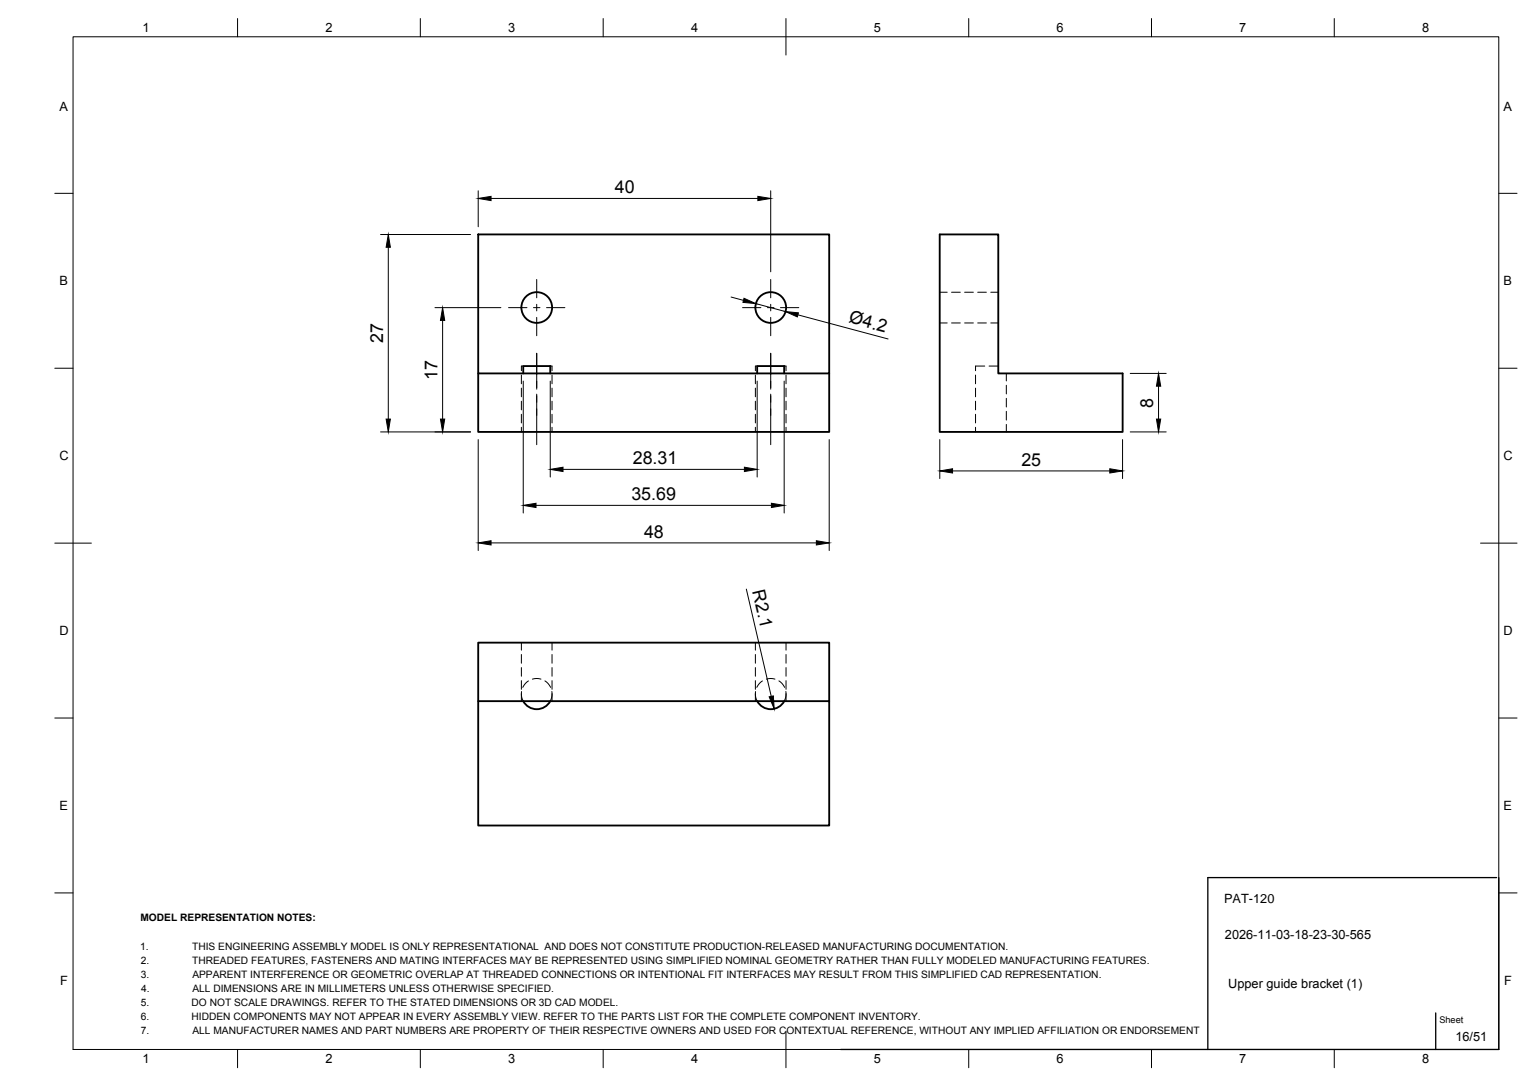
ISO-10303-21;
HEADER;
/* Generated by software containing ST-Developer
 * from STEP Tools, Inc. (www.steptools.com) 
 */

FILE_DESCRIPTION(
/* description */ ('Vibration shaker table dummy'),
/* implementation_level */ '2;1');

FILE_NAME(
/* name */ 'Upper guide bracket (1).step',
/* time_stamp */ '2026-10-27T10:55:14-07:00',
/* author */ (''),
/* organization */ (''),
/* preprocessor_version */ 'ST-DEVELOPER v20.2',
/* originating_system */ 'Autodesk Translation Framework v15.17.0.0',
/* authorisation */ '');

FILE_SCHEMA (('AUTOMOTIVE_DESIGN { 1 0 10303 214 3 1 1 }'));
ENDSEC;

DATA;
#10=MECHANICAL_DESIGN_GEOMETRIC_PRESENTATION_REPRESENTATION('',(#697),#22394);
#605=SHAPE_REPRESENTATION_RELATIONSHIP('SRR','None',#22651,#651);
#651=ADVANCED_BREP_SHAPE_REPRESENTATION('',(#743),#22357);
#697=STYLED_ITEM('',(#22940),#743);
#743=MANIFOLD_SOLID_BREP('Body1',#9215);
#883=FACE_BOUND('',#2092,.T.);
#884=FACE_BOUND('',#2093,.T.);
#885=FACE_BOUND('',#2097,.T.);
#886=FACE_BOUND('',#2098,.T.);
#887=FACE_BOUND('',#2101,.T.);
#888=FACE_BOUND('',#2102,.T.);
#1134=PLANE('',#10051);
#1135=PLANE('',#10057);
#1136=PLANE('',#10058);
#1137=PLANE('',#10059);
#1138=PLANE('',#10060);
#1139=PLANE('',#10061);
#1140=PLANE('',#10062);
#1141=PLANE('',#10063);
#1142=PLANE('',#10064);
#1143=PLANE('',#10065);
#1478=FACE_OUTER_BOUND('',#2084,.T.);
#1479=FACE_OUTER_BOUND('',#2085,.T.);
#1480=FACE_OUTER_BOUND('',#2086,.T.);
#1481=FACE_OUTER_BOUND('',#2087,.T.);
#1482=FACE_OUTER_BOUND('',#2088,.T.);
#1483=FACE_OUTER_BOUND('',#2089,.T.);
#1484=FACE_OUTER_BOUND('',#2090,.T.);
#1485=FACE_OUTER_BOUND('',#2091,.T.);
#1486=FACE_OUTER_BOUND('',#2094,.T.);
#1487=FACE_OUTER_BOUND('',#2095,.T.);
#1488=FACE_OUTER_BOUND('',#2096,.T.);
#1489=FACE_OUTER_BOUND('',#2099,.T.);
#1490=FACE_OUTER_BOUND('',#2100,.T.);
#1491=FACE_OUTER_BOUND('',#2103,.T.);
#2084=EDGE_LOOP('',(#6876,#6877,#6878,#6879));
#2085=EDGE_LOOP('',(#6880,#6881,#6882,#6883));
#2086=EDGE_LOOP('',(#6884,#6885,#6886,#6887,#6888,#6889,#6890,#6891));
#2087=EDGE_LOOP('',(#6892,#6893,#6894));
#2088=EDGE_LOOP('',(#6895,#6896,#6897,#6898,#6899,#6900,#6901,#6902));
#2089=EDGE_LOOP('',(#6903,#6904,#6905));
#2090=EDGE_LOOP('',(#6906,#6907,#6908,#6909,#6910,#6911,#6912,#6913));
#2091=EDGE_LOOP('',(#6914,#6915,#6916,#6917,#6918,#6919,#6920,#6921,#6922,
#6923,#6924,#6925));
#2092=EDGE_LOOP('',(#6926));
#2093=EDGE_LOOP('',(#6927));
#2094=EDGE_LOOP('',(#6928,#6929,#6930,#6931));
#2095=EDGE_LOOP('',(#6932,#6933,#6934,#6935,#6936,#6937));
#2096=EDGE_LOOP('',(#6938,#6939,#6940,#6941));
#2097=EDGE_LOOP('',(#6942));
#2098=EDGE_LOOP('',(#6943));
#2099=EDGE_LOOP('',(#6944,#6945,#6946,#6947,#6948,#6949));
#2100=EDGE_LOOP('',(#6950,#6951,#6952,#6953));
#2101=EDGE_LOOP('',(#6954));
#2102=EDGE_LOOP('',(#6955));
#2103=EDGE_LOOP('',(#6956,#6957,#6958,#6959));
#2806=LINE('',#16101,#3425);
#2807=LINE('',#16107,#3426);
#2808=LINE('',#16113,#3427);
#2809=LINE('',#16117,#3428);
#2810=LINE('',#16121,#3429);
#2811=LINE('',#16124,#3430);
#2812=LINE('',#16129,#3431);
#2813=LINE('',#16133,#3432);
#2814=LINE('',#16137,#3433);
#2815=LINE('',#16140,#3434);
#2816=LINE('',#16142,#3435);
#2817=LINE('',#16144,#3436);
#2818=LINE('',#16146,#3437);
#2819=LINE('',#16148,#3438);
#2820=LINE('',#16150,#3439);
#2821=LINE('',#16151,#3440);
#2822=LINE('',#16154,#3441);
#2823=LINE('',#16156,#3442);
#2824=LINE('',#16157,#3443);
#2825=LINE('',#16161,#3444);
#2826=LINE('',#16162,#3445);
#2827=LINE('',#16163,#3446);
#2828=LINE('',#16167,#3447);
#2829=LINE('',#16168,#3448);
#2830=LINE('',#16169,#3449);
#2831=LINE('',#16173,#3450);
#2832=LINE('',#16174,#3451);
#2833=LINE('',#16175,#3452);
#2834=LINE('',#16177,#3453);
#2835=LINE('',#16178,#3454);
#3425=VECTOR('',#11698,0.21);
#3426=VECTOR('',#11705,0.21);
#3427=VECTOR('',#11712,0.21);
#3428=VECTOR('',#11715,1.);
#3429=VECTOR('',#11718,1.);
#3430=VECTOR('',#11723,1.);
#3431=VECTOR('',#11728,0.21);
#3432=VECTOR('',#11731,1.);
#3433=VECTOR('',#11734,1.);
#3434=VECTOR('',#11739,1.);
#3435=VECTOR('',#11742,1.);
#3436=VECTOR('',#11743,1.);
#3437=VECTOR('',#11744,1.);
#3438=VECTOR('',#11745,1.);
#3439=VECTOR('',#11746,1.);
#3440=VECTOR('',#11747,1.);
#3441=VECTOR('',#11750,1.);
#3442=VECTOR('',#11751,1.);
#3443=VECTOR('',#11752,1.);
#3444=VECTOR('',#11755,1.);
#3445=VECTOR('',#11756,1.);
#3446=VECTOR('',#11757,1.);
#3447=VECTOR('',#11760,1.);
#3448=VECTOR('',#11761,1.);
#3449=VECTOR('',#11762,1.);
#3450=VECTOR('',#11765,1.);
#3451=VECTOR('',#11766,1.);
#3452=VECTOR('',#11767,1.);
#3453=VECTOR('',#11770,1.);
#3454=VECTOR('',#11771,1.);
#3990=CIRCLE('',#10041,0.21);
#3991=CIRCLE('',#10042,0.21);
#3992=CIRCLE('',#10044,0.21);
#3993=CIRCLE('',#10045,0.21);
#3994=CIRCLE('',#10047,0.21);
#3995=CIRCLE('',#10048,0.21);
#3996=CIRCLE('',#10049,0.21);
#3997=CIRCLE('',#10050,0.21);
#3998=CIRCLE('',#10053,0.21);
#3999=CIRCLE('',#10054,0.21);
#4000=CIRCLE('',#10055,0.21);
#4001=CIRCLE('',#10056,0.21);
#4577=VERTEX_POINT('',#16098);
#4578=VERTEX_POINT('',#16100);
#4579=VERTEX_POINT('',#16104);
#4580=VERTEX_POINT('',#16106);
#4581=VERTEX_POINT('',#16110);
#4582=VERTEX_POINT('',#16112);
#4583=VERTEX_POINT('',#16114);
#4584=VERTEX_POINT('',#16116);
#4585=VERTEX_POINT('',#16118);
#4586=VERTEX_POINT('',#16120);
#4587=VERTEX_POINT('',#16126);
#4588=VERTEX_POINT('',#16128);
#4589=VERTEX_POINT('',#16130);
#4590=VERTEX_POINT('',#16132);
#4591=VERTEX_POINT('',#16134);
#4592=VERTEX_POINT('',#16136);
#4593=VERTEX_POINT('',#16143);
#4594=VERTEX_POINT('',#16145);
#4595=VERTEX_POINT('',#16147);
#4596=VERTEX_POINT('',#16149);
#4597=VERTEX_POINT('',#16153);
#4598=VERTEX_POINT('',#16155);
#4599=VERTEX_POINT('',#16159);
#4600=VERTEX_POINT('',#16160);
#4601=VERTEX_POINT('',#16165);
#4602=VERTEX_POINT('',#16166);
#4603=VERTEX_POINT('',#16171);
#4604=VERTEX_POINT('',#16172);
#5431=EDGE_CURVE('',#4577,#4577,#3990,.T.);
#5432=EDGE_CURVE('',#4577,#4578,#2806,.T.);
#5433=EDGE_CURVE('',#4578,#4578,#3991,.T.);
#5434=EDGE_CURVE('',#4579,#4579,#3992,.T.);
#5435=EDGE_CURVE('',#4579,#4580,#2807,.T.);
#5436=EDGE_CURVE('',#4580,#4580,#3993,.T.);
#5437=EDGE_CURVE('',#4581,#4581,#3994,.T.);
#5438=EDGE_CURVE('',#4581,#4582,#2808,.T.);
#5439=EDGE_CURVE('',#4582,#4583,#3995,.T.);
#5440=EDGE_CURVE('',#4584,#4583,#2809,.T.);
#5441=EDGE_CURVE('',#4585,#4584,#3996,.T.);
#5442=EDGE_CURVE('',#4586,#4585,#2810,.T.);
#5443=EDGE_CURVE('',#4586,#4582,#3997,.T.);
#5444=EDGE_CURVE('',#4583,#4586,#2811,.T.);
#5445=EDGE_CURVE('',#4587,#4587,#3998,.T.);
#5446=EDGE_CURVE('',#4587,#4588,#2812,.T.);
#5447=EDGE_CURVE('',#4588,#4589,#3999,.T.);
#5448=EDGE_CURVE('',#4590,#4589,#2813,.T.);
#5449=EDGE_CURVE('',#4591,#4590,#4000,.T.);
#5450=EDGE_CURVE('',#4592,#4591,#2814,.T.);
#5451=EDGE_CURVE('',#4592,#4588,#4001,.T.);
#5452=EDGE_CURVE('',#4589,#4592,#2815,.T.);
#5453=EDGE_CURVE('',#4584,#4591,#2816,.T.);
#5454=EDGE_CURVE('',#4590,#4593,#2817,.T.);
#5455=EDGE_CURVE('',#4594,#4593,#2818,.T.);
#5456=EDGE_CURVE('',#4594,#4595,#2819,.T.);
#5457=EDGE_CURVE('',#4595,#4596,#2820,.T.);
#5458=EDGE_CURVE('',#4596,#4585,#2821,.T.);
#5459=EDGE_CURVE('',#4596,#4597,#2822,.T.);
#5460=EDGE_CURVE('',#4598,#4597,#2823,.T.);
#5461=EDGE_CURVE('',#4593,#4598,#2824,.T.);
#5462=EDGE_CURVE('',#4599,#4600,#2825,.T.);
#5463=EDGE_CURVE('',#4600,#4598,#2826,.T.);
#5464=EDGE_CURVE('',#4597,#4599,#2827,.T.);
#5465=EDGE_CURVE('',#4601,#4602,#2828,.T.);
#5466=EDGE_CURVE('',#4601,#4594,#2829,.T.);
#5467=EDGE_CURVE('',#4602,#4600,#2830,.T.);
#5468=EDGE_CURVE('',#4603,#4604,#2831,.T.);
#5469=EDGE_CURVE('',#4603,#4601,#2832,.T.);
#5470=EDGE_CURVE('',#4604,#4602,#2833,.T.);
#5471=EDGE_CURVE('',#4595,#4603,#2834,.T.);
#5472=EDGE_CURVE('',#4604,#4599,#2835,.T.);
#6876=ORIENTED_EDGE('',*,*,#5431,.F.);
#6877=ORIENTED_EDGE('',*,*,#5432,.T.);
#6878=ORIENTED_EDGE('',*,*,#5433,.F.);
#6879=ORIENTED_EDGE('',*,*,#5432,.F.);
#6880=ORIENTED_EDGE('',*,*,#5434,.F.);
#6881=ORIENTED_EDGE('',*,*,#5435,.T.);
#6882=ORIENTED_EDGE('',*,*,#5436,.F.);
#6883=ORIENTED_EDGE('',*,*,#5435,.F.);
#6884=ORIENTED_EDGE('',*,*,#5437,.F.);
#6885=ORIENTED_EDGE('',*,*,#5438,.T.);
#6886=ORIENTED_EDGE('',*,*,#5439,.T.);
#6887=ORIENTED_EDGE('',*,*,#5440,.F.);
#6888=ORIENTED_EDGE('',*,*,#5441,.F.);
#6889=ORIENTED_EDGE('',*,*,#5442,.F.);
#6890=ORIENTED_EDGE('',*,*,#5443,.T.);
#6891=ORIENTED_EDGE('',*,*,#5438,.F.);
#6892=ORIENTED_EDGE('',*,*,#5444,.F.);
#6893=ORIENTED_EDGE('',*,*,#5439,.F.);
#6894=ORIENTED_EDGE('',*,*,#5443,.F.);
#6895=ORIENTED_EDGE('',*,*,#5445,.F.);
#6896=ORIENTED_EDGE('',*,*,#5446,.T.);
#6897=ORIENTED_EDGE('',*,*,#5447,.T.);
#6898=ORIENTED_EDGE('',*,*,#5448,.F.);
#6899=ORIENTED_EDGE('',*,*,#5449,.F.);
#6900=ORIENTED_EDGE('',*,*,#5450,.F.);
#6901=ORIENTED_EDGE('',*,*,#5451,.T.);
#6902=ORIENTED_EDGE('',*,*,#5446,.F.);
#6903=ORIENTED_EDGE('',*,*,#5452,.F.);
#6904=ORIENTED_EDGE('',*,*,#5447,.F.);
#6905=ORIENTED_EDGE('',*,*,#5451,.F.);
#6906=ORIENTED_EDGE('',*,*,#5441,.T.);
#6907=ORIENTED_EDGE('',*,*,#5453,.T.);
#6908=ORIENTED_EDGE('',*,*,#5449,.T.);
#6909=ORIENTED_EDGE('',*,*,#5454,.T.);
#6910=ORIENTED_EDGE('',*,*,#5455,.F.);
#6911=ORIENTED_EDGE('',*,*,#5456,.T.);
#6912=ORIENTED_EDGE('',*,*,#5457,.T.);
#6913=ORIENTED_EDGE('',*,*,#5458,.T.);
#6914=ORIENTED_EDGE('',*,*,#5442,.T.);
#6915=ORIENTED_EDGE('',*,*,#5458,.F.);
#6916=ORIENTED_EDGE('',*,*,#5459,.T.);
#6917=ORIENTED_EDGE('',*,*,#5460,.F.);
#6918=ORIENTED_EDGE('',*,*,#5461,.F.);
#6919=ORIENTED_EDGE('',*,*,#5454,.F.);
#6920=ORIENTED_EDGE('',*,*,#5448,.T.);
#6921=ORIENTED_EDGE('',*,*,#5452,.T.);
#6922=ORIENTED_EDGE('',*,*,#5450,.T.);
#6923=ORIENTED_EDGE('',*,*,#5453,.F.);
#6924=ORIENTED_EDGE('',*,*,#5440,.T.);
#6925=ORIENTED_EDGE('',*,*,#5444,.T.);
#6926=ORIENTED_EDGE('',*,*,#5431,.T.);
#6927=ORIENTED_EDGE('',*,*,#5434,.T.);
#6928=ORIENTED_EDGE('',*,*,#5462,.T.);
#6929=ORIENTED_EDGE('',*,*,#5463,.T.);
#6930=ORIENTED_EDGE('',*,*,#5460,.T.);
#6931=ORIENTED_EDGE('',*,*,#5464,.T.);
#6932=ORIENTED_EDGE('',*,*,#5465,.F.);
#6933=ORIENTED_EDGE('',*,*,#5466,.T.);
#6934=ORIENTED_EDGE('',*,*,#5455,.T.);
#6935=ORIENTED_EDGE('',*,*,#5461,.T.);
#6936=ORIENTED_EDGE('',*,*,#5463,.F.);
#6937=ORIENTED_EDGE('',*,*,#5467,.F.);
#6938=ORIENTED_EDGE('',*,*,#5468,.F.);
#6939=ORIENTED_EDGE('',*,*,#5469,.T.);
#6940=ORIENTED_EDGE('',*,*,#5465,.T.);
#6941=ORIENTED_EDGE('',*,*,#5470,.F.);
#6942=ORIENTED_EDGE('',*,*,#5437,.T.);
#6943=ORIENTED_EDGE('',*,*,#5445,.T.);
#6944=ORIENTED_EDGE('',*,*,#5457,.F.);
#6945=ORIENTED_EDGE('',*,*,#5471,.T.);
#6946=ORIENTED_EDGE('',*,*,#5468,.T.);
#6947=ORIENTED_EDGE('',*,*,#5472,.T.);
#6948=ORIENTED_EDGE('',*,*,#5464,.F.);
#6949=ORIENTED_EDGE('',*,*,#5459,.F.);
#6950=ORIENTED_EDGE('',*,*,#5472,.F.);
#6951=ORIENTED_EDGE('',*,*,#5470,.T.);
#6952=ORIENTED_EDGE('',*,*,#5467,.T.);
#6953=ORIENTED_EDGE('',*,*,#5462,.F.);
#6954=ORIENTED_EDGE('',*,*,#5433,.T.);
#6955=ORIENTED_EDGE('',*,*,#5436,.T.);
#6956=ORIENTED_EDGE('',*,*,#5471,.F.);
#6957=ORIENTED_EDGE('',*,*,#5456,.F.);
#6958=ORIENTED_EDGE('',*,*,#5466,.F.);
#6959=ORIENTED_EDGE('',*,*,#5469,.F.);
#8568=CYLINDRICAL_SURFACE('',#10040,0.21);
#8569=CYLINDRICAL_SURFACE('',#10043,0.21);
#8570=CYLINDRICAL_SURFACE('',#10046,0.21);
#8571=CYLINDRICAL_SURFACE('',#10052,0.21);
#8843=ADVANCED_FACE('',(#1478),#8568,.F.);
#8844=ADVANCED_FACE('',(#1479),#8569,.F.);
#8845=ADVANCED_FACE('',(#1480),#8570,.F.);
#8846=ADVANCED_FACE('',(#1481),#1134,.F.);
#8847=ADVANCED_FACE('',(#1482),#8571,.F.);
#8848=ADVANCED_FACE('',(#1483),#1135,.F.);
#8849=ADVANCED_FACE('',(#1484),#1136,.T.);
#8850=ADVANCED_FACE('',(#1485,#883,#884),#1137,.T.);
#8851=ADVANCED_FACE('',(#1486),#1138,.T.);
#8852=ADVANCED_FACE('',(#1487),#1139,.T.);
#8853=ADVANCED_FACE('',(#1488,#885,#886),#1140,.T.);
#8854=ADVANCED_FACE('',(#1489),#1141,.T.);
#8855=ADVANCED_FACE('',(#1490,#887,#888),#1142,.T.);
#8856=ADVANCED_FACE('',(#1491),#1143,.F.);
#9215=CLOSED_SHELL('',(#8843,#8844,#8845,#8846,#8847,#8848,#8849,#8850,
#8851,#8852,#8853,#8854,#8855,#8856));
#10039=AXIS2_PLACEMENT_3D('',#16096,#11692,#11693);
#10040=AXIS2_PLACEMENT_3D('',#16097,#11694,#11695);
#10041=AXIS2_PLACEMENT_3D('',#16099,#11696,#11697);
#10042=AXIS2_PLACEMENT_3D('',#16102,#11699,#11700);
#10043=AXIS2_PLACEMENT_3D('',#16103,#11701,#11702);
#10044=AXIS2_PLACEMENT_3D('',#16105,#11703,#11704);
#10045=AXIS2_PLACEMENT_3D('',#16108,#11706,#11707);
#10046=AXIS2_PLACEMENT_3D('',#16109,#11708,#11709);
#10047=AXIS2_PLACEMENT_3D('',#16111,#11710,#11711);
#10048=AXIS2_PLACEMENT_3D('',#16115,#11713,#11714);
#10049=AXIS2_PLACEMENT_3D('',#16119,#11716,#11717);
#10050=AXIS2_PLACEMENT_3D('',#16122,#11719,#11720);
#10051=AXIS2_PLACEMENT_3D('',#16123,#11721,#11722);
#10052=AXIS2_PLACEMENT_3D('',#16125,#11724,#11725);
#10053=AXIS2_PLACEMENT_3D('',#16127,#11726,#11727);
#10054=AXIS2_PLACEMENT_3D('',#16131,#11729,#11730);
#10055=AXIS2_PLACEMENT_3D('',#16135,#11732,#11733);
#10056=AXIS2_PLACEMENT_3D('',#16138,#11735,#11736);
#10057=AXIS2_PLACEMENT_3D('',#16139,#11737,#11738);
#10058=AXIS2_PLACEMENT_3D('',#16141,#11740,#11741);
#10059=AXIS2_PLACEMENT_3D('',#16152,#11748,#11749);
#10060=AXIS2_PLACEMENT_3D('',#16158,#11753,#11754);
#10061=AXIS2_PLACEMENT_3D('',#16164,#11758,#11759);
#10062=AXIS2_PLACEMENT_3D('',#16170,#11763,#11764);
#10063=AXIS2_PLACEMENT_3D('',#16176,#11768,#11769);
#10064=AXIS2_PLACEMENT_3D('',#16179,#11772,#11773);
#10065=AXIS2_PLACEMENT_3D('',#16180,#11774,#11775);
#11692=DIRECTION('axis',(0.,0.,1.));
#11693=DIRECTION('refdir',(1.,0.,0.));
#11694=DIRECTION('center_axis',(0.,0.,1.));
#11695=DIRECTION('ref_axis',(1.,0.,0.));
#11696=DIRECTION('center_axis',(0.,0.,1.));
#11697=DIRECTION('ref_axis',(1.,0.,0.));
#11698=DIRECTION('',(0.,0.,1.));
#11699=DIRECTION('center_axis',(0.,0.,-1.));
#11700=DIRECTION('ref_axis',(1.,0.,0.));
#11701=DIRECTION('center_axis',(0.,0.,1.));
#11702=DIRECTION('ref_axis',(1.,0.,0.));
#11703=DIRECTION('center_axis',(0.,0.,1.));
#11704=DIRECTION('ref_axis',(1.,0.,0.));
#11705=DIRECTION('',(0.,0.,1.));
#11706=DIRECTION('center_axis',(0.,0.,-1.));
#11707=DIRECTION('ref_axis',(1.,0.,0.));
#11708=DIRECTION('center_axis',(0.,1.,0.));
#11709=DIRECTION('ref_axis',(1.,0.,0.));
#11710=DIRECTION('center_axis',(0.,1.,0.));
#11711=DIRECTION('ref_axis',(1.,0.,0.));
#11712=DIRECTION('',(0.,1.,0.));
#11713=DIRECTION('center_axis',(0.,1.,0.));
#11714=DIRECTION('ref_axis',(1.,0.,0.));
#11715=DIRECTION('',(0.,1.,0.));
#11716=DIRECTION('center_axis',(0.,-1.,0.));
#11717=DIRECTION('ref_axis',(1.,0.,0.));
#11718=DIRECTION('',(0.,-1.,0.));
#11719=DIRECTION('center_axis',(0.,1.,0.));
#11720=DIRECTION('ref_axis',(1.,0.,0.));
#11721=DIRECTION('center_axis',(0.,1.,0.));
#11722=DIRECTION('ref_axis',(1.,0.,0.));
#11723=DIRECTION('',(-1.,0.,0.));
#11724=DIRECTION('center_axis',(0.,1.,0.));
#11725=DIRECTION('ref_axis',(1.,0.,0.));
#11726=DIRECTION('center_axis',(0.,1.,0.));
#11727=DIRECTION('ref_axis',(1.,0.,0.));
#11728=DIRECTION('',(0.,1.,0.));
#11729=DIRECTION('center_axis',(0.,1.,0.));
#11730=DIRECTION('ref_axis',(1.,0.,0.));
#11731=DIRECTION('',(0.,1.,0.));
#11732=DIRECTION('center_axis',(0.,-1.,0.));
#11733=DIRECTION('ref_axis',(1.,0.,0.));
#11734=DIRECTION('',(0.,-1.,0.));
#11735=DIRECTION('center_axis',(0.,1.,0.));
#11736=DIRECTION('ref_axis',(1.,0.,0.));
#11737=DIRECTION('center_axis',(0.,1.,0.));
#11738=DIRECTION('ref_axis',(1.,0.,0.));
#11739=DIRECTION('',(-1.,0.,0.));
#11740=DIRECTION('center_axis',(0.,1.,0.));
#11741=DIRECTION('ref_axis',(-1.,0.,0.));
#11742=DIRECTION('',(1.,0.,0.));
#11743=DIRECTION('',(1.,0.,0.));
#11744=DIRECTION('',(0.,0.,1.));
#11745=DIRECTION('',(-1.,0.,0.));
#11746=DIRECTION('',(0.,0.,1.));
#11747=DIRECTION('',(1.,0.,0.));
#11748=DIRECTION('center_axis',(0.,0.,-1.));
#11749=DIRECTION('ref_axis',(-1.,0.,0.));
#11750=DIRECTION('',(0.,1.,0.));
#11751=DIRECTION('',(-1.,0.,0.));
#11752=DIRECTION('',(0.,1.,0.));
#11753=DIRECTION('center_axis',(0.,1.,0.));
#11754=DIRECTION('ref_axis',(0.,0.,1.));
#11755=DIRECTION('',(1.,0.,0.));
#11756=DIRECTION('',(0.,0.,-1.));
#11757=DIRECTION('',(0.,0.,1.));
#11758=DIRECTION('center_axis',(1.,0.,0.));
#11759=DIRECTION('ref_axis',(0.,1.,0.));
#11760=DIRECTION('',(0.,0.,1.));
#11761=DIRECTION('',(0.,1.,0.));
#11762=DIRECTION('',(0.,1.,0.));
#11763=DIRECTION('center_axis',(0.,-1.,0.));
#11764=DIRECTION('ref_axis',(1.,0.,0.));
#11765=DIRECTION('',(0.,0.,1.));
#11766=DIRECTION('',(1.,0.,0.));
#11767=DIRECTION('',(1.,0.,0.));
#11768=DIRECTION('center_axis',(-1.,0.,0.));
#11769=DIRECTION('ref_axis',(0.,-1.,0.));
#11770=DIRECTION('',(0.,-1.,0.));
#11771=DIRECTION('',(0.,1.,0.));
#11772=DIRECTION('center_axis',(0.,0.,1.));
#11773=DIRECTION('ref_axis',(1.,0.,0.));
#11774=DIRECTION('center_axis',(0.,0.,1.));
#11775=DIRECTION('ref_axis',(1.,0.,0.));
#16096=CARTESIAN_POINT('',(0.,0.,0.));
#16097=CARTESIAN_POINT('Origin',(-7.6,8.,29.6));
#16098=CARTESIAN_POINT('',(-7.81,8.,29.7));
#16099=CARTESIAN_POINT('Origin',(-7.6,8.,29.7));
#16100=CARTESIAN_POINT('',(-7.81,8.,30.5));
#16101=CARTESIAN_POINT('',(-7.81,8.,29.6));
#16102=CARTESIAN_POINT('Origin',(-7.6,8.,30.5));
#16103=CARTESIAN_POINT('Origin',(-4.4,8.,29.6));
#16104=CARTESIAN_POINT('',(-4.61,8.,29.7));
#16105=CARTESIAN_POINT('Origin',(-4.4,8.,29.7));
#16106=CARTESIAN_POINT('',(-4.61,8.,30.5));
#16107=CARTESIAN_POINT('',(-4.61,8.,29.6));
#16108=CARTESIAN_POINT('Origin',(-4.4,8.,30.5));
#16109=CARTESIAN_POINT('Origin',(-7.6,6.2,29.8));
#16110=CARTESIAN_POINT('',(-7.81,6.3,29.8));
#16111=CARTESIAN_POINT('Origin',(-7.6,6.3,29.8));
#16112=CARTESIAN_POINT('',(-7.81,7.2,29.8));
#16113=CARTESIAN_POINT('',(-7.81,6.2,29.8));
#16114=CARTESIAN_POINT('',(-7.41533814687381,7.2,29.7));
#16115=CARTESIAN_POINT('Origin',(-7.6,7.2,29.8));
#16116=CARTESIAN_POINT('',(-7.4153381468738,7.1,29.7));
#16117=CARTESIAN_POINT('',(-7.41533814687381,6.2,29.7));
#16118=CARTESIAN_POINT('',(-7.78466185312619,7.1,29.7));
#16119=CARTESIAN_POINT('Origin',(-7.6,7.1,29.8));
#16120=CARTESIAN_POINT('',(-7.78466185312619,7.2,29.7));
#16121=CARTESIAN_POINT('',(-7.78466185312619,6.2,29.7));
#16122=CARTESIAN_POINT('Origin',(-7.6,7.2,29.8));
#16123=CARTESIAN_POINT('Origin',(-7.6,7.2,29.8));
#16124=CARTESIAN_POINT('',(-5.6,7.2,29.7));
#16125=CARTESIAN_POINT('Origin',(-4.4,6.2,29.8));
#16126=CARTESIAN_POINT('',(-4.61,6.3,29.8));
#16127=CARTESIAN_POINT('Origin',(-4.4,6.3,29.8));
#16128=CARTESIAN_POINT('',(-4.61,7.2,29.8));
#16129=CARTESIAN_POINT('',(-4.61,6.2,29.8));
#16130=CARTESIAN_POINT('',(-4.21533814687381,7.2,29.7));
#16131=CARTESIAN_POINT('Origin',(-4.4,7.2,29.8));
#16132=CARTESIAN_POINT('',(-4.21533814687381,7.1,29.7));
#16133=CARTESIAN_POINT('',(-4.21533814687381,6.2,29.7));
#16134=CARTESIAN_POINT('',(-4.5846618531262,7.1,29.7));
#16135=CARTESIAN_POINT('Origin',(-4.4,7.1,29.8));
#16136=CARTESIAN_POINT('',(-4.58466185312619,7.2,29.7));
#16137=CARTESIAN_POINT('',(-4.58466185312619,6.2,29.7));
#16138=CARTESIAN_POINT('Origin',(-4.4,7.2,29.8));
#16139=CARTESIAN_POINT('Origin',(-4.4,7.2,29.8));
#16140=CARTESIAN_POINT('',(-4.,7.2,29.7));
#16141=CARTESIAN_POINT('Origin',(-3.6,7.1,28.));
#16142=CARTESIAN_POINT('',(-3.6,7.1,29.7));
#16143=CARTESIAN_POINT('',(-3.6,7.1,29.7));
#16144=CARTESIAN_POINT('',(-3.6,7.1,29.7));
#16145=CARTESIAN_POINT('',(-3.6,7.1,28.));
#16146=CARTESIAN_POINT('',(-3.6,7.1,28.));
#16147=CARTESIAN_POINT('',(-8.4,7.1,28.));
#16148=CARTESIAN_POINT('',(-3.6,7.1,28.));
#16149=CARTESIAN_POINT('',(-8.4,7.1,29.7));
#16150=CARTESIAN_POINT('',(-8.4,7.1,28.));
#16151=CARTESIAN_POINT('',(-3.6,7.1,29.7));
#16152=CARTESIAN_POINT('Origin',(-3.6,6.3,29.7));
#16153=CARTESIAN_POINT('',(-8.4,9.,29.7));
#16154=CARTESIAN_POINT('',(-8.4,6.3,29.7));
#16155=CARTESIAN_POINT('',(-3.6,9.,29.7));
#16156=CARTESIAN_POINT('',(-8.4,9.,29.7));
#16157=CARTESIAN_POINT('',(-3.6,6.3,29.7));
#16158=CARTESIAN_POINT('Origin',(-6.,9.,30.1));
#16159=CARTESIAN_POINT('',(-8.4,9.,30.5));
#16160=CARTESIAN_POINT('',(-3.6,9.,30.5));
#16161=CARTESIAN_POINT('',(-3.6,9.,30.5));
#16162=CARTESIAN_POINT('',(-3.6,9.,29.7));
#16163=CARTESIAN_POINT('',(-8.4,9.,30.5));
#16164=CARTESIAN_POINT('Origin',(-3.6,6.3,28.));
#16165=CARTESIAN_POINT('',(-3.6,6.3,28.));
#16166=CARTESIAN_POINT('',(-3.6,6.3,30.5));
#16167=CARTESIAN_POINT('',(-3.6,6.3,28.));
#16168=CARTESIAN_POINT('',(-3.6,6.3,28.));
#16169=CARTESIAN_POINT('',(-3.6,6.3,30.5));
#16170=CARTESIAN_POINT('Origin',(-8.4,6.3,28.));
#16171=CARTESIAN_POINT('',(-8.4,6.3,28.));
#16172=CARTESIAN_POINT('',(-8.4,6.3,30.5));
#16173=CARTESIAN_POINT('',(-8.4,6.3,28.));
#16174=CARTESIAN_POINT('',(-8.4,6.3,28.));
#16175=CARTESIAN_POINT('',(-8.4,6.3,30.5));
#16176=CARTESIAN_POINT('Origin',(-8.4,7.1,28.));
#16177=CARTESIAN_POINT('',(-8.4,7.1,28.));
#16178=CARTESIAN_POINT('',(-8.4,6.3,30.5));
#16179=CARTESIAN_POINT('Origin',(-6.,6.7,30.5));
#16180=CARTESIAN_POINT('Origin',(-6.,6.7,28.));
#22306=UNCERTAINTY_MEASURE_WITH_UNIT(LENGTH_MEASURE(0.001),#22395,
'DISTANCE_ACCURACY_VALUE',
'Maximum model space distance between geometric entities at asserted c
onnectivities');
#22343=UNCERTAINTY_MEASURE_WITH_UNIT(LENGTH_MEASURE(0.001),#22395,
'DISTANCE_ACCURACY_VALUE',
'Maximum model space distance between geometric entities at asserted c
onnectivities');
#22357=(
GEOMETRIC_REPRESENTATION_CONTEXT(3)
GLOBAL_UNCERTAINTY_ASSIGNED_CONTEXT((#22306))
GLOBAL_UNIT_ASSIGNED_CONTEXT((#22395,#22397,#22398))
REPRESENTATION_CONTEXT('','3D')
);
#22394=(
GEOMETRIC_REPRESENTATION_CONTEXT(3)
GLOBAL_UNCERTAINTY_ASSIGNED_CONTEXT((#22343))
GLOBAL_UNIT_ASSIGNED_CONTEXT((#22395,#22397,#22398))
REPRESENTATION_CONTEXT('','3D')
);
#22395=(
LENGTH_UNIT()
NAMED_UNIT(*)
SI_UNIT(.CENTI.,.METRE.)
);
#22397=(
NAMED_UNIT(*)
PLANE_ANGLE_UNIT()
SI_UNIT($,.RADIAN.)
);
#22398=(
NAMED_UNIT(*)
SI_UNIT($,.STERADIAN.)
SOLID_ANGLE_UNIT()
);
#22412=SHAPE_DEFINITION_REPRESENTATION(#22462,#22651);
#22462=PRODUCT_DEFINITION_SHAPE('',$,#22702);
#22651=SHAPE_REPRESENTATION('',(#10039),#22357);
#22688=PRODUCT_DEFINITION_CONTEXT('part definition',#22840,'design');
#22702=PRODUCT_DEFINITION('Upper guide bracket (1)',
'Upper guide bracket (1)',#22752,#22688);
#22752=PRODUCT_DEFINITION_FORMATION('',$,#22855);
#22840=APPLICATION_CONTEXT(
'Core Data for Automotive Mechanical Design Process');
#22841=PRODUCT_CONTEXT('part definition',#22840,'mechanical');
#22855=PRODUCT('Upper guide bracket (1)','Upper guide bracket (1)',
'Upper guide bracket (1)',(#22841));
#22934=COLOUR_RGB('Dark Blue',0.08,0.2,0.34);
#22935=FILL_AREA_STYLE_COLOUR('',#22934);
#22936=FILL_AREA_STYLE('',(#22935));
#22937=SURFACE_STYLE_FILL_AREA(#22936);
#22938=SURFACE_SIDE_STYLE('',(#22937));
#22939=SURFACE_STYLE_USAGE(.BOTH.,#22938);
#22940=PRESENTATION_STYLE_ASSIGNMENT((#22939));
ENDSEC;
END-ISO-10303-21;
